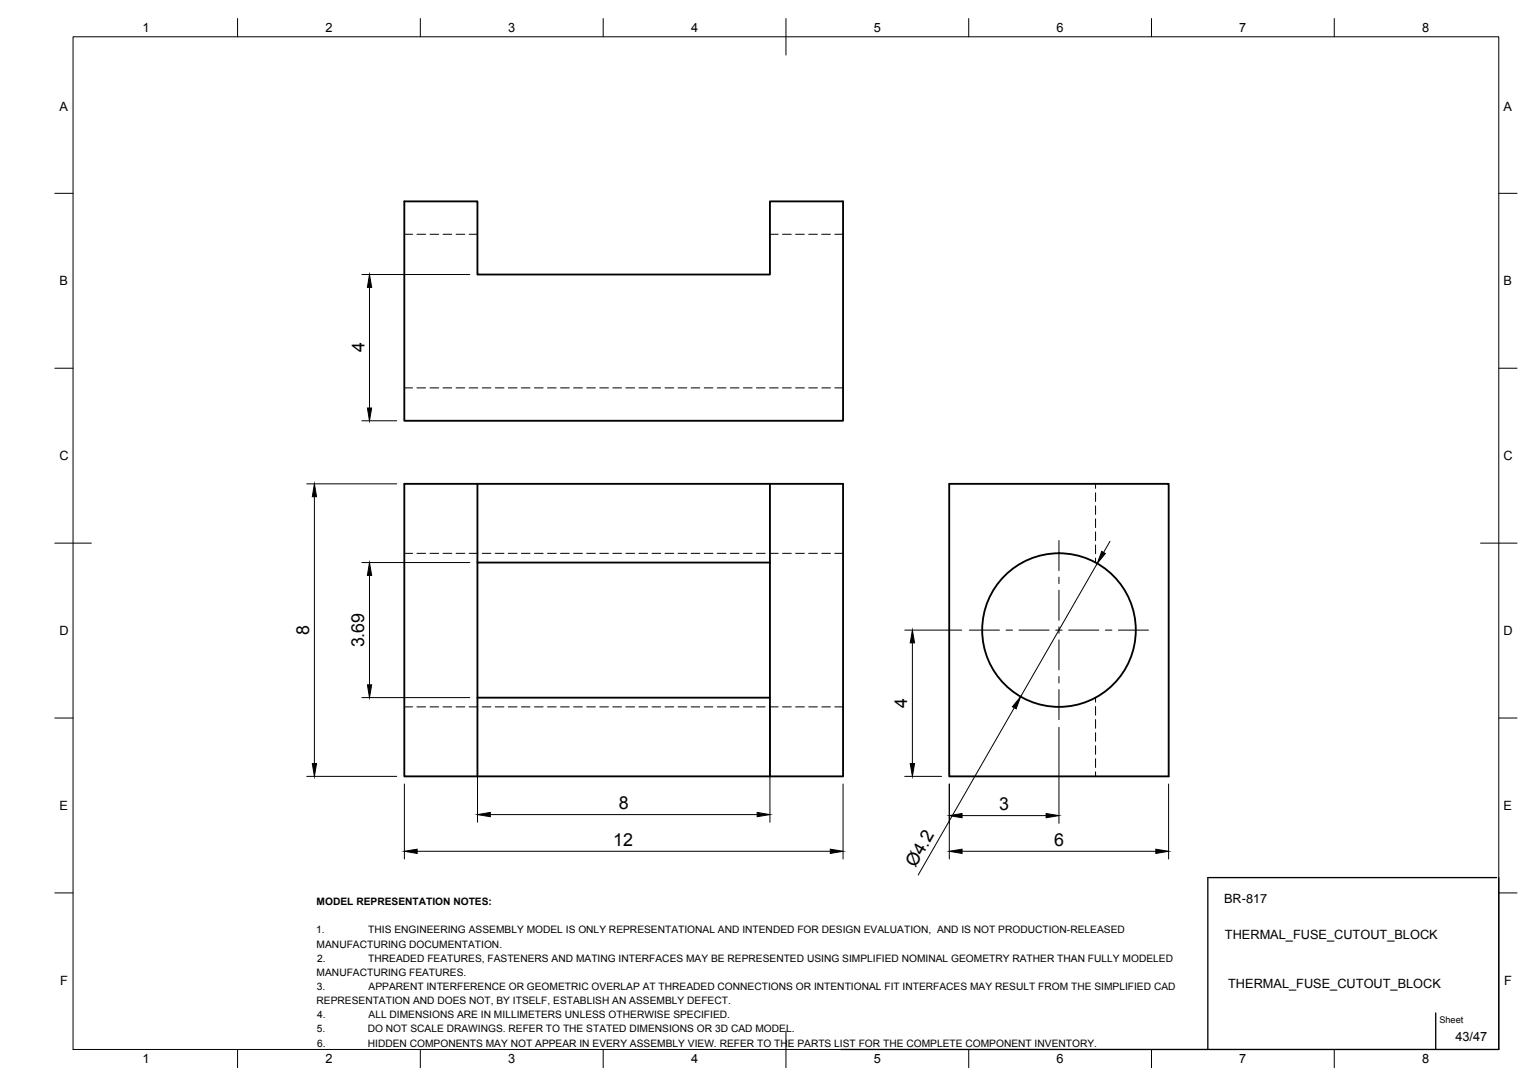
ISO-10303-21;
HEADER;
FILE_DESCRIPTION((''),'2;1');
FILE_NAME('THERMAL_FUSE_CUTOUT_BLOCK.step','2026-10-01T22:07:29-07:00',(''),(''),'','','');
FILE_SCHEMA (('AUTOMOTIVE_DESIGN { 1 0 10303 214 3 1 1 }'));
ENDSEC;
DATA;
#10=MECHANICAL_DESIGN_GEOMETRIC_PRESENTATION_REPRESENTATION('',(#578),#15484);
#503=SHAPE_REPRESENTATION_RELATIONSHIP('SRR','None',#15654,#538) ;
#538=ADVANCED_BREP_SHAPE_REPRESENTATION('',(#619),#15478) ;
#578=STYLED_ITEM('',(#15833),#619) ;
#619=MANIFOLD_SOLID_BREP('THERMAL_FUSE_CUTOUT_BLOCK',#8289) ;
#801=CYLINDRICAL_SURFACE('',#9856,0.21) ;
#881=FACE_BOUND('',#2413,.T.) ;
#882=FACE_BOUND('',#2415,.T.) ;
#1343=CIRCLE('',#9846,0.21) ;
#1344=CIRCLE('',#9847,0.21) ;
#1345=CIRCLE('',#9851,0.21) ;
#1346=CIRCLE('',#9852,0.21) ;
#1347=CIRCLE('',#9857,0.21) ;
#1348=CIRCLE('',#9858,0.21) ;
#1831=FACE_OUTER_BOUND('',#2402,.T.) ;
#1832=FACE_OUTER_BOUND('',#2403,.T.) ;
#1833=FACE_OUTER_BOUND('',#2404,.T.) ;
#1834=FACE_OUTER_BOUND('',#2405,.T.) ;
#1835=FACE_OUTER_BOUND('',#2406,.T.) ;
#1836=FACE_OUTER_BOUND('',#2407,.T.) ;
#1837=FACE_OUTER_BOUND('',#2408,.T.) ;
#1838=FACE_OUTER_BOUND('',#2409,.T.) ;
#1839=FACE_OUTER_BOUND('',#2410,.T.) ;
#1840=FACE_OUTER_BOUND('',#2411,.T.) ;
#1841=FACE_OUTER_BOUND('',#2412,.T.) ;
#1842=FACE_OUTER_BOUND('',#2414,.T.) ;
#2402=EDGE_LOOP('',(#7417,#7418,#7419,#7420,#7421,#7422,#7423)) ;
#2403=EDGE_LOOP('',(#7424,#7425,#7426,#7427)) ;
#2404=EDGE_LOOP('',(#7428,#7429,#7430,#7431)) ;
#2405=EDGE_LOOP('',(#7432,#7433,#7434,#7435,#7436,#7437,#7438)) ;
#2406=EDGE_LOOP('',(#7439,#7440,#7441,#7442,#7443,#7444,#7445,#7446)) ;
#2407=EDGE_LOOP('',(#7447,#7448,#7449,#7450)) ;
#2408=EDGE_LOOP('',(#7451,#7452,#7453,#7454)) ;
#2409=EDGE_LOOP('',(#7455,#7456,#7457,#7458,#7459,#7460,#7461,#7462,#7463,
#7464,#7465,#7466)) ;
#2410=EDGE_LOOP('',(#7467,#7468,#7469,#7470)) ;
#2411=EDGE_LOOP('',(#7471,#7472,#7473,#7474,#7475,#7476,#7477,#7478)) ;
#2412=EDGE_LOOP('',(#7479,#7480,#7481,#7482)) ;
#2413=EDGE_LOOP('',(#7483)) ;
#2414=EDGE_LOOP('',(#7484,#7485,#7486,#7487)) ;
#2415=EDGE_LOOP('',(#7488)) ;
#2876=LINE('',#15246,#3350) ;
#2877=LINE('',#15248,#3351) ;
#2878=LINE('',#15250,#3352) ;
#2879=LINE('',#15252,#3353) ;
#2880=LINE('',#15254,#3354) ;
#2881=LINE('',#15258,#3355) ;
#2882=LINE('',#15260,#3356) ;
#2883=LINE('',#15261,#3357) ;
#2884=LINE('',#15264,#3358) ;
#2885=LINE('',#15266,#3359) ;
#2886=LINE('',#15267,#3360) ;
#2887=LINE('',#15272,#3361) ;
#2888=LINE('',#15274,#3362) ;
#2889=LINE('',#15275,#3363) ;
#2890=LINE('',#15279,#3364) ;
#2891=LINE('',#15281,#3365) ;
#2892=LINE('',#15283,#3366) ;
#2893=LINE('',#15285,#3367) ;
#2894=LINE('',#15286,#3368) ;
#2895=LINE('',#15289,#3369) ;
#2896=LINE('',#15290,#3370) ;
#2897=LINE('',#15293,#3371) ;
#2898=LINE('',#15294,#3372) ;
#2899=LINE('',#15298,#3373) ;
#2900=LINE('',#15300,#3374) ;
#2901=LINE('',#15304,#3375) ;
#2902=LINE('',#15306,#3376) ;
#2903=LINE('',#15307,#3377) ;
#2904=LINE('',#15309,#3378) ;
#2905=LINE('',#15310,#3379) ;
#3350=VECTOR('',#12691,1.) ;
#3351=VECTOR('',#12692,1.) ;
#3352=VECTOR('',#12693,1.) ;
#3353=VECTOR('',#12694,1.) ;
#3354=VECTOR('',#12695,1.) ;
#3355=VECTOR('',#12700,1.) ;
#3356=VECTOR('',#12701,1.) ;
#3357=VECTOR('',#12702,1.) ;
#3358=VECTOR('',#12705,1.) ;
#3359=VECTOR('',#12706,1.) ;
#3360=VECTOR('',#12707,1.) ;
#3361=VECTOR('',#12712,1.) ;
#3362=VECTOR('',#12713,1.) ;
#3363=VECTOR('',#12714,1.) ;
#3364=VECTOR('',#12719,1.) ;
#3365=VECTOR('',#12720,1.) ;
#3366=VECTOR('',#12721,1.) ;
#3367=VECTOR('',#12722,1.) ;
#3368=VECTOR('',#12723,1.) ;
#3369=VECTOR('',#12726,1.) ;
#3370=VECTOR('',#12727,1.) ;
#3371=VECTOR('',#12730,1.) ;
#3372=VECTOR('',#12731,1.) ;
#3373=VECTOR('',#12736,0.21) ;
#3374=VECTOR('',#12737,0.21) ;
#3375=VECTOR('',#12742,1.) ;
#3376=VECTOR('',#12743,1.) ;
#3377=VECTOR('',#12744,1.) ;
#3378=VECTOR('',#12747,1.) ;
#3379=VECTOR('',#12748,1.) ;
#4101=VERTEX_POINT('',#15242) ;
#4102=VERTEX_POINT('',#15243) ;
#4103=VERTEX_POINT('',#15245) ;
#4104=VERTEX_POINT('',#15247) ;
#4105=VERTEX_POINT('',#15249) ;
#4106=VERTEX_POINT('',#15251) ;
#4107=VERTEX_POINT('',#15253) ;
#4108=VERTEX_POINT('',#15257) ;
#4109=VERTEX_POINT('',#15259) ;
#4110=VERTEX_POINT('',#15263) ;
#4111=VERTEX_POINT('',#15265) ;
#4112=VERTEX_POINT('',#15269) ;
#4113=VERTEX_POINT('',#15271) ;
#4114=VERTEX_POINT('',#15273) ;
#4115=VERTEX_POINT('',#15278) ;
#4116=VERTEX_POINT('',#15280) ;
#4117=VERTEX_POINT('',#15282) ;
#4118=VERTEX_POINT('',#15284) ;
#4119=VERTEX_POINT('',#15288) ;
#4120=VERTEX_POINT('',#15292) ;
#4121=VERTEX_POINT('',#15296) ;
#4122=VERTEX_POINT('',#15299) ;
#4123=VERTEX_POINT('',#15303) ;
#4124=VERTEX_POINT('',#15305) ;
#5213=EDGE_CURVE('',#4101,#4102,#1343,.T.) ;
#5214=EDGE_CURVE('',#4101,#4103,#2876,.T.) ;
#5215=EDGE_CURVE('',#4104,#4103,#2877,.T.) ;
#5216=EDGE_CURVE('',#4105,#4104,#2878,.T.) ;
#5217=EDGE_CURVE('',#4106,#4105,#2879,.T.) ;
#5218=EDGE_CURVE('',#4106,#4107,#2880,.T.) ;
#5219=EDGE_CURVE('',#4102,#4107,#1344,.T.) ;
#5220=EDGE_CURVE('',#4107,#4108,#2881,.T.) ;
#5221=EDGE_CURVE('',#4109,#4106,#2882,.T.) ;
#5222=EDGE_CURVE('',#4108,#4109,#2883,.T.) ;
#5223=EDGE_CURVE('',#4110,#4101,#2884,.T.) ;
#5224=EDGE_CURVE('',#4111,#4110,#2885,.T.) ;
#5225=EDGE_CURVE('',#4103,#4111,#2886,.T.) ;
#5226=EDGE_CURVE('',#4108,#4112,#1345,.T.) ;
#5227=EDGE_CURVE('',#4113,#4109,#2887,.T.) ;
#5228=EDGE_CURVE('',#4114,#4113,#2888,.T.) ;
#5229=EDGE_CURVE('',#4111,#4114,#2889,.T.) ;
#5230=EDGE_CURVE('',#4112,#4110,#1346,.T.) ;
#5231=EDGE_CURVE('',#4115,#4114,#2890,.T.) ;
#5232=EDGE_CURVE('',#4115,#4116,#2891,.T.) ;
#5233=EDGE_CURVE('',#4117,#4116,#2892,.T.) ;
#5234=EDGE_CURVE('',#4118,#4117,#2893,.T.) ;
#5235=EDGE_CURVE('',#4104,#4118,#2894,.T.) ;
#5236=EDGE_CURVE('',#4113,#4119,#2895,.T.) ;
#5237=EDGE_CURVE('',#4119,#4115,#2896,.T.) ;
#5238=EDGE_CURVE('',#4118,#4120,#2897,.T.) ;
#5239=EDGE_CURVE('',#4120,#4105,#2898,.T.) ;
#5240=EDGE_CURVE('',#4121,#4121,#1347,.T.) ;
#5241=EDGE_CURVE('',#4121,#4102,#2899,.T.) ;
#5242=EDGE_CURVE('',#4112,#4122,#2900,.T.) ;
#5243=EDGE_CURVE('',#4122,#4122,#1348,.T.) ;
#5244=EDGE_CURVE('',#4116,#4123,#2901,.T.) ;
#5245=EDGE_CURVE('',#4123,#4124,#2902,.T.) ;
#5246=EDGE_CURVE('',#4124,#4117,#2903,.T.) ;
#5247=EDGE_CURVE('',#4120,#4124,#2904,.T.) ;
#5248=EDGE_CURVE('',#4119,#4123,#2905,.T.) ;
#7417=ORIENTED_EDGE('',*,*,#5213,.F.) ;
#7418=ORIENTED_EDGE('',*,*,#5214,.T.) ;
#7419=ORIENTED_EDGE('',*,*,#5215,.F.) ;
#7420=ORIENTED_EDGE('',*,*,#5216,.F.) ;
#7421=ORIENTED_EDGE('',*,*,#5217,.F.) ;
#7422=ORIENTED_EDGE('',*,*,#5218,.T.) ;
#7423=ORIENTED_EDGE('',*,*,#5219,.F.) ;
#7424=ORIENTED_EDGE('',*,*,#5220,.F.) ;
#7425=ORIENTED_EDGE('',*,*,#5218,.F.) ;
#7426=ORIENTED_EDGE('',*,*,#5221,.F.) ;
#7427=ORIENTED_EDGE('',*,*,#5222,.F.) ;
#7428=ORIENTED_EDGE('',*,*,#5223,.F.) ;
#7429=ORIENTED_EDGE('',*,*,#5224,.F.) ;
#7430=ORIENTED_EDGE('',*,*,#5225,.F.) ;
#7431=ORIENTED_EDGE('',*,*,#5214,.F.) ;
#7432=ORIENTED_EDGE('',*,*,#5226,.F.) ;
#7433=ORIENTED_EDGE('',*,*,#5222,.T.) ;
#7434=ORIENTED_EDGE('',*,*,#5227,.F.) ;
#7435=ORIENTED_EDGE('',*,*,#5228,.F.) ;
#7436=ORIENTED_EDGE('',*,*,#5229,.F.) ;
#7437=ORIENTED_EDGE('',*,*,#5224,.T.) ;
#7438=ORIENTED_EDGE('',*,*,#5230,.F.) ;
#7439=ORIENTED_EDGE('',*,*,#5215,.T.) ;
#7440=ORIENTED_EDGE('',*,*,#5225,.T.) ;
#7441=ORIENTED_EDGE('',*,*,#5229,.T.) ;
#7442=ORIENTED_EDGE('',*,*,#5231,.F.) ;
#7443=ORIENTED_EDGE('',*,*,#5232,.T.) ;
#7444=ORIENTED_EDGE('',*,*,#5233,.F.) ;
#7445=ORIENTED_EDGE('',*,*,#5234,.F.) ;
#7446=ORIENTED_EDGE('',*,*,#5235,.F.) ;
#7447=ORIENTED_EDGE('',*,*,#5228,.T.) ;
#7448=ORIENTED_EDGE('',*,*,#5236,.T.) ;
#7449=ORIENTED_EDGE('',*,*,#5237,.T.) ;
#7450=ORIENTED_EDGE('',*,*,#5231,.T.) ;
#7451=ORIENTED_EDGE('',*,*,#5216,.T.) ;
#7452=ORIENTED_EDGE('',*,*,#5235,.T.) ;
#7453=ORIENTED_EDGE('',*,*,#5238,.T.) ;
#7454=ORIENTED_EDGE('',*,*,#5239,.T.) ;
#7455=ORIENTED_EDGE('',*,*,#5240,.F.) ;
#7456=ORIENTED_EDGE('',*,*,#5241,.T.) ;
#7457=ORIENTED_EDGE('',*,*,#5219,.T.) ;
#7458=ORIENTED_EDGE('',*,*,#5220,.T.) ;
#7459=ORIENTED_EDGE('',*,*,#5226,.T.) ;
#7460=ORIENTED_EDGE('',*,*,#5242,.T.) ;
#7461=ORIENTED_EDGE('',*,*,#5243,.F.) ;
#7462=ORIENTED_EDGE('',*,*,#5242,.F.) ;
#7463=ORIENTED_EDGE('',*,*,#5230,.T.) ;
#7464=ORIENTED_EDGE('',*,*,#5223,.T.) ;
#7465=ORIENTED_EDGE('',*,*,#5213,.T.) ;
#7466=ORIENTED_EDGE('',*,*,#5241,.F.) ;
#7467=ORIENTED_EDGE('',*,*,#5244,.T.) ;
#7468=ORIENTED_EDGE('',*,*,#5245,.T.) ;
#7469=ORIENTED_EDGE('',*,*,#5246,.T.) ;
#7470=ORIENTED_EDGE('',*,*,#5233,.T.) ;
#7471=ORIENTED_EDGE('',*,*,#5217,.T.) ;
#7472=ORIENTED_EDGE('',*,*,#5239,.F.) ;
#7473=ORIENTED_EDGE('',*,*,#5247,.T.) ;
#7474=ORIENTED_EDGE('',*,*,#5245,.F.) ;
#7475=ORIENTED_EDGE('',*,*,#5248,.F.) ;
#7476=ORIENTED_EDGE('',*,*,#5236,.F.) ;
#7477=ORIENTED_EDGE('',*,*,#5227,.T.) ;
#7478=ORIENTED_EDGE('',*,*,#5221,.T.) ;
#7479=ORIENTED_EDGE('',*,*,#5234,.T.) ;
#7480=ORIENTED_EDGE('',*,*,#5246,.F.) ;
#7481=ORIENTED_EDGE('',*,*,#5247,.F.) ;
#7482=ORIENTED_EDGE('',*,*,#5238,.F.) ;
#7483=ORIENTED_EDGE('',*,*,#5240,.T.) ;
#7484=ORIENTED_EDGE('',*,*,#5248,.T.) ;
#7485=ORIENTED_EDGE('',*,*,#5244,.F.) ;
#7486=ORIENTED_EDGE('',*,*,#5232,.F.) ;
#7487=ORIENTED_EDGE('',*,*,#5237,.F.) ;
#7488=ORIENTED_EDGE('',*,*,#5243,.T.) ;
#7727=PLANE('',#9845) ;
#7728=PLANE('',#9848) ;
#7729=PLANE('',#9849) ;
#7730=PLANE('',#9850) ;
#7731=PLANE('',#9853) ;
#7732=PLANE('',#9854) ;
#7733=PLANE('',#9855) ;
#7734=PLANE('',#9859) ;
#7735=PLANE('',#9860) ;
#7736=PLANE('',#9861) ;
#7737=PLANE('',#9862) ;
#8218=ADVANCED_FACE('',(#1831),#7727,.T.) ;
#8219=ADVANCED_FACE('',(#1832),#7728,.T.) ;
#8220=ADVANCED_FACE('',(#1833),#7729,.T.) ;
#8221=ADVANCED_FACE('',(#1834),#7730,.T.) ;
#8222=ADVANCED_FACE('',(#1835),#7731,.F.) ;
#8223=ADVANCED_FACE('',(#1836),#7732,.T.) ;
#8224=ADVANCED_FACE('',(#1837),#7733,.T.) ;
#8225=ADVANCED_FACE('',(#1838),#801,.F.) ;
#8226=ADVANCED_FACE('',(#1839),#7734,.F.) ;
#8227=ADVANCED_FACE('',(#1840),#7735,.F.) ;
#8228=ADVANCED_FACE('',(#1841,#881),#7736,.F.) ;
#8229=ADVANCED_FACE('',(#1842,#882),#7737,.F.) ;
#8289=CLOSED_SHELL('',(#8218,#8219,#8220,#8221,#8222,#8223,#8224,#8225,
#8226,#8227,#8228,#8229)) ;
#9844=AXIS2_PLACEMENT_3D('',#15240,#12685,#12686) ;
#9845=AXIS2_PLACEMENT_3D('',#15241,#12687,#12688) ;
#9846=AXIS2_PLACEMENT_3D('',#15244,#12689,#12690) ;
#9847=AXIS2_PLACEMENT_3D('',#15255,#12696,#12697) ;
#9848=AXIS2_PLACEMENT_3D('',#15256,#12698,#12699) ;
#9849=AXIS2_PLACEMENT_3D('',#15262,#12703,#12704) ;
#9850=AXIS2_PLACEMENT_3D('',#15268,#12708,#12709) ;
#9851=AXIS2_PLACEMENT_3D('',#15270,#12710,#12711) ;
#9852=AXIS2_PLACEMENT_3D('',#15276,#12715,#12716) ;
#9853=AXIS2_PLACEMENT_3D('',#15277,#12717,#12718) ;
#9854=AXIS2_PLACEMENT_3D('',#15287,#12724,#12725) ;
#9855=AXIS2_PLACEMENT_3D('',#15291,#12728,#12729) ;
#9856=AXIS2_PLACEMENT_3D('',#15295,#12732,#12733) ;
#9857=AXIS2_PLACEMENT_3D('',#15297,#12734,#12735) ;
#9858=AXIS2_PLACEMENT_3D('',#15301,#12738,#12739) ;
#9859=AXIS2_PLACEMENT_3D('',#15302,#12740,#12741) ;
#9860=AXIS2_PLACEMENT_3D('',#15308,#12745,#12746) ;
#9861=AXIS2_PLACEMENT_3D('',#15311,#12749,#12750) ;
#9862=AXIS2_PLACEMENT_3D('',#15312,#12751,#12752) ;
#12685=DIRECTION('axis',(0.,0.,1.)) ;
#12686=DIRECTION('refdir',(1.,0.,0.)) ;
#12687=DIRECTION('center_axis',(1.,0.,0.)) ;
#12688=DIRECTION('ref_axis',(0.,0.,-1.)) ;
#12689=DIRECTION('center_axis',(1.,0.,0.)) ;
#12690=DIRECTION('ref_axis',(0.,0.,-1.)) ;
#12691=DIRECTION('',(0.,1.,0.)) ;
#12692=DIRECTION('',(0.,0.,-1.)) ;
#12693=DIRECTION('',(0.,1.,0.)) ;
#12694=DIRECTION('',(0.,0.,1.)) ;
#12695=DIRECTION('',(0.,1.,0.)) ;
#12696=DIRECTION('center_axis',(1.,0.,0.)) ;
#12697=DIRECTION('ref_axis',(0.,0.,-1.)) ;
#12698=DIRECTION('center_axis',(0.,0.,1.)) ;
#12699=DIRECTION('ref_axis',(1.,0.,0.)) ;
#12700=DIRECTION('',(1.,0.,0.)) ;
#12701=DIRECTION('',(-1.,0.,0.)) ;
#12702=DIRECTION('',(0.,-1.,0.)) ;
#12703=DIRECTION('center_axis',(0.,0.,1.)) ;
#12704=DIRECTION('ref_axis',(1.,0.,0.)) ;
#12705=DIRECTION('',(-1.,0.,0.)) ;
#12706=DIRECTION('',(0.,-1.,0.)) ;
#12707=DIRECTION('',(1.,0.,0.)) ;
#12708=DIRECTION('center_axis',(-1.,0.,0.)) ;
#12709=DIRECTION('ref_axis',(0.,0.,1.)) ;
#12710=DIRECTION('center_axis',(-1.,0.,0.)) ;
#12711=DIRECTION('ref_axis',(0.,0.,-1.)) ;
#12712=DIRECTION('',(0.,0.,-1.)) ;
#12713=DIRECTION('',(0.,-1.,0.)) ;
#12714=DIRECTION('',(0.,0.,1.)) ;
#12715=DIRECTION('center_axis',(-1.,0.,0.)) ;
#12716=DIRECTION('ref_axis',(0.,0.,-1.)) ;
#12717=DIRECTION('center_axis',(0.,-1.,0.)) ;
#12718=DIRECTION('ref_axis',(0.,0.,-1.)) ;
#12719=DIRECTION('',(-1.,0.,0.)) ;
#12720=DIRECTION('',(0.,0.,-1.)) ;
#12721=DIRECTION('',(1.,0.,0.)) ;
#12722=DIRECTION('',(0.,0.,-1.)) ;
#12723=DIRECTION('',(-1.,0.,0.)) ;
#12724=DIRECTION('center_axis',(0.,0.,1.)) ;
#12725=DIRECTION('ref_axis',(1.,0.,0.)) ;
#12726=DIRECTION('',(1.,0.,0.)) ;
#12727=DIRECTION('',(0.,1.,0.)) ;
#12728=DIRECTION('center_axis',(0.,0.,1.)) ;
#12729=DIRECTION('ref_axis',(1.,0.,0.)) ;
#12730=DIRECTION('',(0.,-1.,0.)) ;
#12731=DIRECTION('',(1.,0.,0.)) ;
#12732=DIRECTION('center_axis',(1.,0.,0.)) ;
#12733=DIRECTION('ref_axis',(0.,0.,-1.)) ;
#12734=DIRECTION('center_axis',(1.,0.,0.)) ;
#12735=DIRECTION('ref_axis',(0.,0.,-1.)) ;
#12736=DIRECTION('',(1.,0.,0.)) ;
#12737=DIRECTION('',(1.,0.,0.)) ;
#12738=DIRECTION('center_axis',(-1.,0.,0.)) ;
#12739=DIRECTION('ref_axis',(0.,0.,-1.)) ;
#12740=DIRECTION('center_axis',(0.,0.,1.)) ;
#12741=DIRECTION('ref_axis',(1.,0.,0.)) ;
#12742=DIRECTION('',(0.,-1.,0.)) ;
#12743=DIRECTION('',(-1.,0.,0.)) ;
#12744=DIRECTION('',(0.,1.,0.)) ;
#12745=DIRECTION('center_axis',(0.,1.,0.)) ;
#12746=DIRECTION('ref_axis',(0.,0.,1.)) ;
#12747=DIRECTION('',(0.,0.,-1.)) ;
#12748=DIRECTION('',(0.,0.,-1.)) ;
#12749=DIRECTION('center_axis',(1.,0.,0.)) ;
#12750=DIRECTION('ref_axis',(0.,0.,-1.)) ;
#12751=DIRECTION('center_axis',(-1.,0.,0.)) ;
#12752=DIRECTION('ref_axis',(0.,0.,1.)) ;
#15240=CARTESIAN_POINT('',(0.,0.,0.)) ;
#15241=CARTESIAN_POINT('Origin',(1.2,-1.8,0.85)) ;
#15242=CARTESIAN_POINT('',(1.2,-1.61533814687381,0.7)) ;
#15243=CARTESIAN_POINT('',(1.2,-1.8,0.81)) ;
#15244=CARTESIAN_POINT('Origin',(1.2,-1.8,0.6)) ;
#15245=CARTESIAN_POINT('',(1.2,-1.4,0.7)) ;
#15246=CARTESIAN_POINT('',(1.2,-1.8,0.7)) ;
#15247=CARTESIAN_POINT('',(1.2,-1.4,0.9)) ;
#15248=CARTESIAN_POINT('',(1.2,-1.4,0.725)) ;
#15249=CARTESIAN_POINT('',(1.2,-2.2,0.9)) ;
#15250=CARTESIAN_POINT('',(1.2,-1.8,0.9)) ;
#15251=CARTESIAN_POINT('',(1.2,-2.2,0.7)) ;
#15252=CARTESIAN_POINT('',(1.2,-2.2,0.725)) ;
#15253=CARTESIAN_POINT('',(1.2,-1.98466185312619,0.7)) ;
#15254=CARTESIAN_POINT('',(1.2,-1.8,0.7)) ;
#15255=CARTESIAN_POINT('Origin',(1.2,-1.8,0.6)) ;
#15256=CARTESIAN_POINT('Origin',(1.6,-1.8,0.7)) ;
#15257=CARTESIAN_POINT('',(2.,-1.98466185312619,0.7)) ;
#15258=CARTESIAN_POINT('',(1.6,-1.98466185312619,0.7)) ;
#15259=CARTESIAN_POINT('',(2.,-2.2,0.7)) ;
#15260=CARTESIAN_POINT('',(1.6,-2.2,0.7)) ;
#15261=CARTESIAN_POINT('',(2.,-1.8,0.7)) ;
#15262=CARTESIAN_POINT('Origin',(1.6,-1.8,0.7)) ;
#15263=CARTESIAN_POINT('',(2.,-1.61533814687381,0.7)) ;
#15264=CARTESIAN_POINT('',(1.6,-1.61533814687381,0.7)) ;
#15265=CARTESIAN_POINT('',(2.,-1.4,0.7)) ;
#15266=CARTESIAN_POINT('',(2.,-1.8,0.7)) ;
#15267=CARTESIAN_POINT('',(1.6,-1.4,0.7)) ;
#15268=CARTESIAN_POINT('Origin',(2.,-1.8,0.85)) ;
#15269=CARTESIAN_POINT('',(2.,-1.8,0.81)) ;
#15270=CARTESIAN_POINT('Origin',(2.,-1.8,0.6)) ;
#15271=CARTESIAN_POINT('',(2.,-2.2,0.9)) ;
#15272=CARTESIAN_POINT('',(2.,-2.2,0.725)) ;
#15273=CARTESIAN_POINT('',(2.,-1.4,0.9)) ;
#15274=CARTESIAN_POINT('',(2.,-1.8,0.9)) ;
#15275=CARTESIAN_POINT('',(2.,-1.4,0.725)) ;
#15276=CARTESIAN_POINT('Origin',(2.,-1.8,0.6)) ;
#15277=CARTESIAN_POINT('Origin',(1.6,-1.4,0.6)) ;
#15278=CARTESIAN_POINT('',(2.2,-1.4,0.9)) ;
#15279=CARTESIAN_POINT('',(1.6,-1.4,0.9)) ;
#15280=CARTESIAN_POINT('',(2.2,-1.4,0.3)) ;
#15281=CARTESIAN_POINT('',(2.2,-1.4,0.6)) ;
#15282=CARTESIAN_POINT('',(1.,-1.4,0.3)) ;
#15283=CARTESIAN_POINT('',(1.6,-1.4,0.3)) ;
#15284=CARTESIAN_POINT('',(1.,-1.4,0.9)) ;
#15285=CARTESIAN_POINT('',(1.,-1.4,0.6)) ;
#15286=CARTESIAN_POINT('',(1.6,-1.4,0.9)) ;
#15287=CARTESIAN_POINT('Origin',(1.6,-1.8,0.9)) ;
#15288=CARTESIAN_POINT('',(2.2,-2.2,0.9)) ;
#15289=CARTESIAN_POINT('',(1.6,-2.2,0.9)) ;
#15290=CARTESIAN_POINT('',(2.2,-1.8,0.9)) ;
#15291=CARTESIAN_POINT('Origin',(1.6,-1.8,0.9)) ;
#15292=CARTESIAN_POINT('',(1.,-2.2,0.9)) ;
#15293=CARTESIAN_POINT('',(1.,-1.8,0.9)) ;
#15294=CARTESIAN_POINT('',(1.6,-2.2,0.9)) ;
#15295=CARTESIAN_POINT('Origin',(1.6,-1.8,0.6)) ;
#15296=CARTESIAN_POINT('',(1.,-1.8,0.81)) ;
#15297=CARTESIAN_POINT('Origin',(1.,-1.8,0.6)) ;
#15298=CARTESIAN_POINT('',(1.6,-1.8,0.81)) ;
#15299=CARTESIAN_POINT('',(2.2,-1.8,0.81)) ;
#15300=CARTESIAN_POINT('',(1.6,-1.8,0.81)) ;
#15301=CARTESIAN_POINT('Origin',(2.2,-1.8,0.6)) ;
#15302=CARTESIAN_POINT('Origin',(1.6,-1.8,0.3)) ;
#15303=CARTESIAN_POINT('',(2.2,-2.2,0.3)) ;
#15304=CARTESIAN_POINT('',(2.2,-1.8,0.3)) ;
#15305=CARTESIAN_POINT('',(1.,-2.2,0.3)) ;
#15306=CARTESIAN_POINT('',(1.6,-2.2,0.3)) ;
#15307=CARTESIAN_POINT('',(1.,-1.8,0.3)) ;
#15308=CARTESIAN_POINT('Origin',(1.6,-2.2,0.6)) ;
#15309=CARTESIAN_POINT('',(1.,-2.2,0.6)) ;
#15310=CARTESIAN_POINT('',(2.2,-2.2,0.6)) ;
#15311=CARTESIAN_POINT('Origin',(1.,-1.8,0.6)) ;
#15312=CARTESIAN_POINT('Origin',(2.2,-1.8,0.6)) ;
#15435=UNCERTAINTY_MEASURE_WITH_UNIT(LENGTH_MEASURE(0.001),#15485,
'DISTANCE_ACCURACY_VALUE',
'Maximum model space distance between geometric entities at asserted c
onnectivities') ;
#15441=UNCERTAINTY_MEASURE_WITH_UNIT(LENGTH_MEASURE(0.001),#15485,
'DISTANCE_ACCURACY_VALUE',
'Maximum model space distance between geometric entities at asserted c
onnectivities') ;
#15478=(
GEOMETRIC_REPRESENTATION_CONTEXT(3)
GLOBAL_UNCERTAINTY_ASSIGNED_CONTEXT((#15435))
GLOBAL_UNIT_ASSIGNED_CONTEXT((#15485,#15487,#15488))
REPRESENTATION_CONTEXT('','3D')
) ;
#15484=(
GEOMETRIC_REPRESENTATION_CONTEXT(3)
GLOBAL_UNCERTAINTY_ASSIGNED_CONTEXT((#15441))
GLOBAL_UNIT_ASSIGNED_CONTEXT((#15485,#15487,#15488))
REPRESENTATION_CONTEXT('','3D')
) ;
#15485=(
LENGTH_UNIT()
NAMED_UNIT(*)
SI_UNIT(.CENTI.,.METRE.)
) ;
#15487=(
NAMED_UNIT(*)
PLANE_ANGLE_UNIT()
SI_UNIT($,.RADIAN.)
) ;
#15488=(
NAMED_UNIT(*)
SI_UNIT($,.STERADIAN.)
SOLID_ANGLE_UNIT()
) ;
#15525=SHAPE_DEFINITION_REPRESENTATION(#15593,#15654) ;
#15593=PRODUCT_DEFINITION_SHAPE('',$,#15697) ;
#15654=SHAPE_REPRESENTATION('',(#9844),#15478) ;
#15660=PRODUCT_DEFINITION_CONTEXT('part definition',#15788,'design') ;
#15697=PRODUCT_DEFINITION('THERMAL_FUSE_CUTOUT_BLOCK',
'THERMAL_FUSE_CUTOUT_BLOCK',#15739,#15660) ;
#15739=PRODUCT_DEFINITION_FORMATION('',$,#15826) ;
#15788=APPLICATION_CONTEXT(
'Core Data for Automotive Mechanical Design Process') ;
#15789=PRODUCT_CONTEXT('part definition',#15788,'mechanical') ;
#15826=PRODUCT('THERMAL_FUSE_CUTOUT_BLOCK','THERMAL_FUSE_CUTOUT_BLOCK',$,
(#15789)) ;
#15833=PRESENTATION_STYLE_ASSIGNMENT((#15845)) ;
#15845=SURFACE_STYLE_USAGE(.BOTH.,#15857) ;
#15857=SURFACE_SIDE_STYLE('',(#15869)) ;
#15869=SURFACE_STYLE_FILL_AREA(#15881) ;
#15881=FILL_AREA_STYLE('Nylon 6-6 (White)',(#15893)) ;
#15893=FILL_AREA_STYLE_COLOUR('Nylon 6-6 (White)',#15905) ;
#15905=COLOUR_RGB('Nylon 6-6 (White)', 0.31764706, 0.68627451, 0.89019608) ;
ENDSEC;
END-ISO-10303-21;
